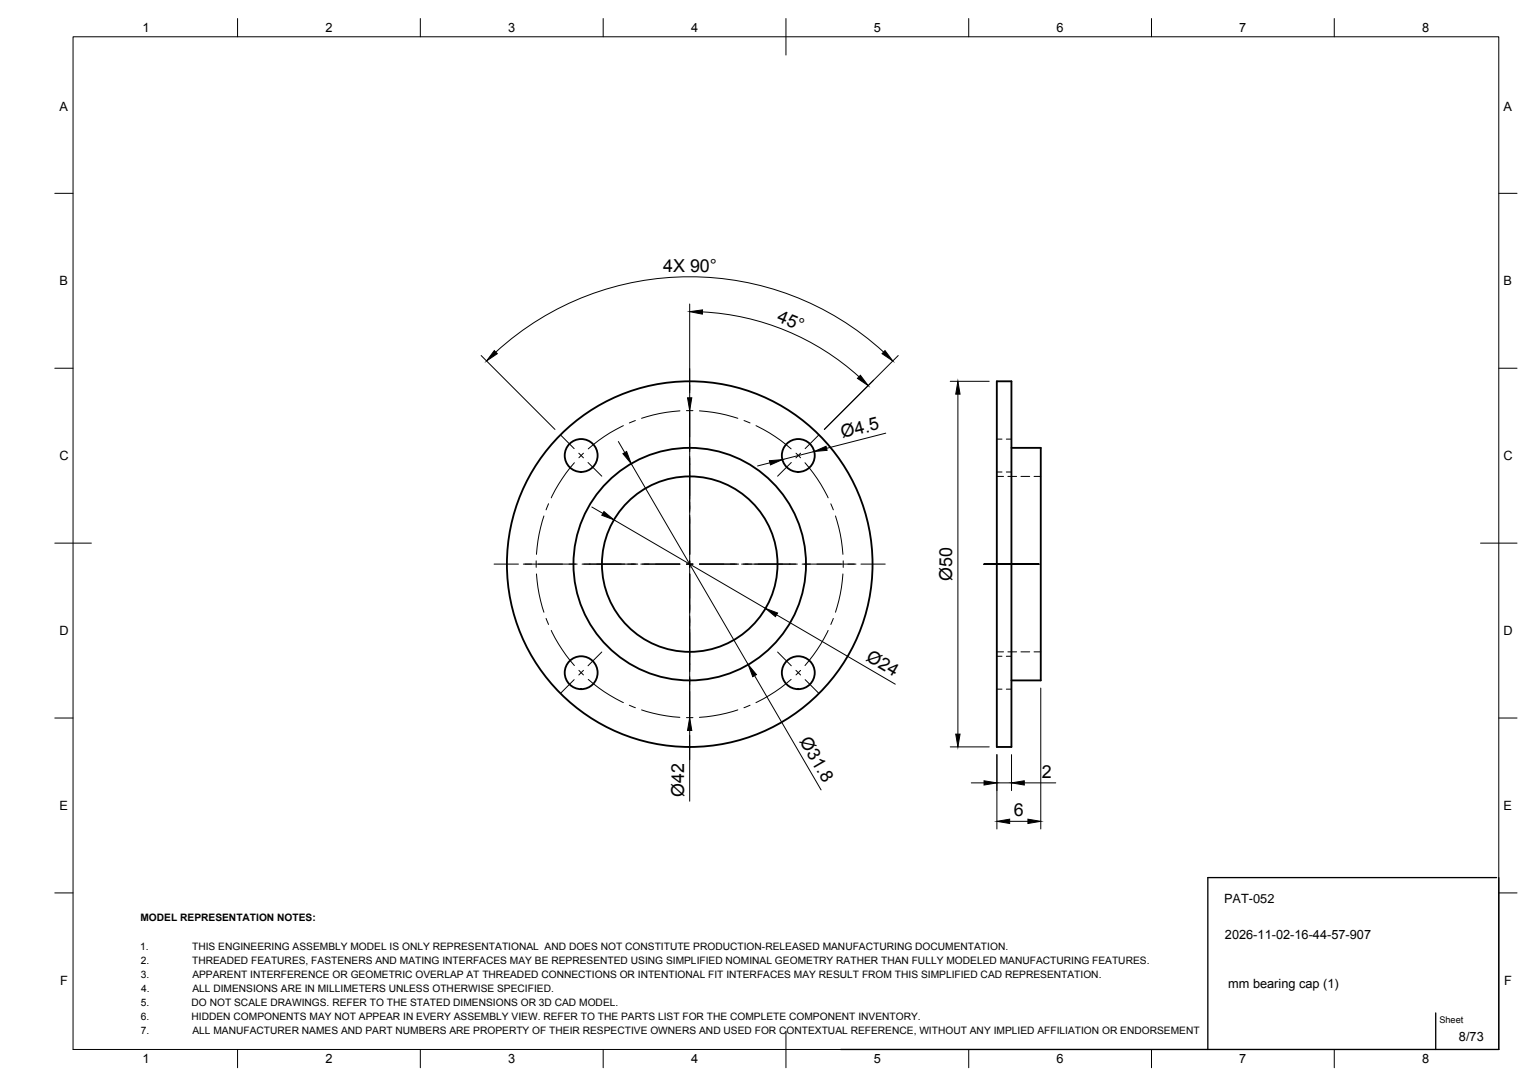
ISO-10303-21;
HEADER;
/* Generated by software containing ST-Developer
 * from STEP Tools, Inc. (www.steptools.com) 
 */

FILE_DESCRIPTION(
/* description */ ('Hand-crank gear train demonstrator'),
/* implementation_level */ '2;1');

FILE_NAME(
/* name */ 'mm bearing cap (1).step',
/* time_stamp */ '2026-10-28T03:22:13-07:00',
/* author */ (''),
/* organization */ (''),
/* preprocessor_version */ 'ST-DEVELOPER v20.2',
/* originating_system */ 'Autodesk Translation Framework v15.17.0.0',
/* authorisation */ '');

FILE_SCHEMA (('AUTOMOTIVE_DESIGN { 1 0 10303 214 3 1 1 }'));
ENDSEC;

DATA;
#10=MECHANICAL_DESIGN_GEOMETRIC_PRESENTATION_REPRESENTATION('',(#1192),#62758);
#1064=SHAPE_REPRESENTATION_RELATIONSHIP('SRR','None',#63036,#1128);
#1128=ADVANCED_BREP_SHAPE_REPRESENTATION('',(#1271),#62690);
#1192=STYLED_ITEM('',(#63462),#1271);
#1271=MANIFOLD_SOLID_BREP('Body1',#16372);
#1409=FACE_BOUND('',#3184,.T.);
#1410=FACE_BOUND('',#3188,.T.);
#1411=FACE_BOUND('',#3189,.T.);
#1412=FACE_BOUND('',#3190,.T.);
#1413=FACE_BOUND('',#3191,.T.);
#1414=FACE_BOUND('',#3192,.T.);
#1415=FACE_BOUND('',#3194,.T.);
#1416=FACE_BOUND('',#3195,.T.);
#1417=FACE_BOUND('',#3196,.T.);
#1418=FACE_BOUND('',#3197,.T.);
#1419=FACE_BOUND('',#3198,.T.);
#1650=PLANE('',#17301);
#1651=PLANE('',#17308);
#1652=PLANE('',#17309);
#2175=FACE_OUTER_BOUND('',#3178,.T.);
#2176=FACE_OUTER_BOUND('',#3179,.T.);
#2177=FACE_OUTER_BOUND('',#3180,.T.);
#2178=FACE_OUTER_BOUND('',#3181,.T.);
#2179=FACE_OUTER_BOUND('',#3182,.T.);
#2180=FACE_OUTER_BOUND('',#3183,.T.);
#2181=FACE_OUTER_BOUND('',#3185,.T.);
#2182=FACE_OUTER_BOUND('',#3186,.T.);
#2183=FACE_OUTER_BOUND('',#3187,.T.);
#2184=FACE_OUTER_BOUND('',#3193,.T.);
#3178=EDGE_LOOP('',(#11105,#11106,#11107,#11108));
#3179=EDGE_LOOP('',(#11109,#11110,#11111,#11112));
#3180=EDGE_LOOP('',(#11113,#11114,#11115,#11116));
#3181=EDGE_LOOP('',(#11117,#11118,#11119,#11120));
#3182=EDGE_LOOP('',(#11121,#11122,#11123,#11124));
#3183=EDGE_LOOP('',(#11125));
#3184=EDGE_LOOP('',(#11126));
#3185=EDGE_LOOP('',(#11127,#11128,#11129,#11130));
#3186=EDGE_LOOP('',(#11131,#11132,#11133,#11134));
#3187=EDGE_LOOP('',(#11135));
#3188=EDGE_LOOP('',(#11136));
#3189=EDGE_LOOP('',(#11137));
#3190=EDGE_LOOP('',(#11138));
#3191=EDGE_LOOP('',(#11139));
#3192=EDGE_LOOP('',(#11140));
#3193=EDGE_LOOP('',(#11141));
#3194=EDGE_LOOP('',(#11142));
#3195=EDGE_LOOP('',(#11143));
#3196=EDGE_LOOP('',(#11144));
#3197=EDGE_LOOP('',(#11145));
#3198=EDGE_LOOP('',(#11146));
#4351=LINE('',#23596,#5483);
#4352=LINE('',#23602,#5484);
#4353=LINE('',#23608,#5485);
#4354=LINE('',#23614,#5486);
#4355=LINE('',#23620,#5487);
#4356=LINE('',#23628,#5488);
#4357=LINE('',#23633,#5489);
#5483=VECTOR('',#19156,0.225);
#5484=VECTOR('',#19163,0.225);
#5485=VECTOR('',#19170,0.225);
#5486=VECTOR('',#19177,0.225);
#5487=VECTOR('',#19184,1.59);
#5488=VECTOR('',#19195,1.2);
#5489=VECTOR('',#19200,2.5);
#6620=CIRCLE('',#17287,0.225);
#6621=CIRCLE('',#17288,0.225);
#6622=CIRCLE('',#17290,0.225);
#6623=CIRCLE('',#17291,0.225);
#6624=CIRCLE('',#17293,0.225);
#6625=CIRCLE('',#17294,0.225);
#6626=CIRCLE('',#17296,0.225);
#6627=CIRCLE('',#17297,0.225);
#6628=CIRCLE('',#17299,1.59);
#6629=CIRCLE('',#17300,1.59);
#6630=CIRCLE('',#17302,1.2);
#6631=CIRCLE('',#17304,1.2);
#6632=CIRCLE('',#17306,2.5);
#6633=CIRCLE('',#17307,2.5);
#7302=VERTEX_POINT('',#23593);
#7303=VERTEX_POINT('',#23595);
#7304=VERTEX_POINT('',#23599);
#7305=VERTEX_POINT('',#23601);
#7306=VERTEX_POINT('',#23605);
#7307=VERTEX_POINT('',#23607);
#7308=VERTEX_POINT('',#23611);
#7309=VERTEX_POINT('',#23613);
#7310=VERTEX_POINT('',#23617);
#7311=VERTEX_POINT('',#23619);
#7312=VERTEX_POINT('',#23623);
#7313=VERTEX_POINT('',#23626);
#7314=VERTEX_POINT('',#23630);
#7315=VERTEX_POINT('',#23632);
#8804=EDGE_CURVE('',#7302,#7302,#6620,.T.);
#8805=EDGE_CURVE('',#7302,#7303,#4351,.T.);
#8806=EDGE_CURVE('',#7303,#7303,#6621,.T.);
#8807=EDGE_CURVE('',#7304,#7304,#6622,.T.);
#8808=EDGE_CURVE('',#7304,#7305,#4352,.T.);
#8809=EDGE_CURVE('',#7305,#7305,#6623,.T.);
#8810=EDGE_CURVE('',#7306,#7306,#6624,.T.);
#8811=EDGE_CURVE('',#7306,#7307,#4353,.T.);
#8812=EDGE_CURVE('',#7307,#7307,#6625,.T.);
#8813=EDGE_CURVE('',#7308,#7308,#6626,.T.);
#8814=EDGE_CURVE('',#7308,#7309,#4354,.T.);
#8815=EDGE_CURVE('',#7309,#7309,#6627,.T.);
#8816=EDGE_CURVE('',#7310,#7310,#6628,.T.);
#8817=EDGE_CURVE('',#7310,#7311,#4355,.T.);
#8818=EDGE_CURVE('',#7311,#7311,#6629,.T.);
#8819=EDGE_CURVE('',#7312,#7312,#6630,.T.);
#8820=EDGE_CURVE('',#7313,#7313,#6631,.T.);
#8821=EDGE_CURVE('',#7313,#7312,#4356,.T.);
#8822=EDGE_CURVE('',#7314,#7314,#6632,.T.);
#8823=EDGE_CURVE('',#7314,#7315,#4357,.T.);
#8824=EDGE_CURVE('',#7315,#7315,#6633,.T.);
#11105=ORIENTED_EDGE('',*,*,#8804,.F.);
#11106=ORIENTED_EDGE('',*,*,#8805,.T.);
#11107=ORIENTED_EDGE('',*,*,#8806,.F.);
#11108=ORIENTED_EDGE('',*,*,#8805,.F.);
#11109=ORIENTED_EDGE('',*,*,#8807,.F.);
#11110=ORIENTED_EDGE('',*,*,#8808,.T.);
#11111=ORIENTED_EDGE('',*,*,#8809,.F.);
#11112=ORIENTED_EDGE('',*,*,#8808,.F.);
#11113=ORIENTED_EDGE('',*,*,#8810,.F.);
#11114=ORIENTED_EDGE('',*,*,#8811,.T.);
#11115=ORIENTED_EDGE('',*,*,#8812,.F.);
#11116=ORIENTED_EDGE('',*,*,#8811,.F.);
#11117=ORIENTED_EDGE('',*,*,#8813,.F.);
#11118=ORIENTED_EDGE('',*,*,#8814,.T.);
#11119=ORIENTED_EDGE('',*,*,#8815,.F.);
#11120=ORIENTED_EDGE('',*,*,#8814,.F.);
#11121=ORIENTED_EDGE('',*,*,#8816,.F.);
#11122=ORIENTED_EDGE('',*,*,#8817,.T.);
#11123=ORIENTED_EDGE('',*,*,#8818,.T.);
#11124=ORIENTED_EDGE('',*,*,#8817,.F.);
#11125=ORIENTED_EDGE('',*,*,#8818,.F.);
#11126=ORIENTED_EDGE('',*,*,#8819,.F.);
#11127=ORIENTED_EDGE('',*,*,#8820,.F.);
#11128=ORIENTED_EDGE('',*,*,#8821,.T.);
#11129=ORIENTED_EDGE('',*,*,#8819,.T.);
#11130=ORIENTED_EDGE('',*,*,#8821,.F.);
#11131=ORIENTED_EDGE('',*,*,#8822,.F.);
#11132=ORIENTED_EDGE('',*,*,#8823,.T.);
#11133=ORIENTED_EDGE('',*,*,#8824,.T.);
#11134=ORIENTED_EDGE('',*,*,#8823,.F.);
#11135=ORIENTED_EDGE('',*,*,#8822,.T.);
#11136=ORIENTED_EDGE('',*,*,#8820,.T.);
#11137=ORIENTED_EDGE('',*,*,#8815,.T.);
#11138=ORIENTED_EDGE('',*,*,#8812,.T.);
#11139=ORIENTED_EDGE('',*,*,#8809,.T.);
#11140=ORIENTED_EDGE('',*,*,#8806,.T.);
#11141=ORIENTED_EDGE('',*,*,#8824,.F.);
#11142=ORIENTED_EDGE('',*,*,#8816,.T.);
#11143=ORIENTED_EDGE('',*,*,#8813,.T.);
#11144=ORIENTED_EDGE('',*,*,#8810,.T.);
#11145=ORIENTED_EDGE('',*,*,#8807,.T.);
#11146=ORIENTED_EDGE('',*,*,#8804,.T.);
#15202=CYLINDRICAL_SURFACE('',#17286,0.225);
#15203=CYLINDRICAL_SURFACE('',#17289,0.225);
#15204=CYLINDRICAL_SURFACE('',#17292,0.225);
#15205=CYLINDRICAL_SURFACE('',#17295,0.225);
#15206=CYLINDRICAL_SURFACE('',#17298,1.59);
#15207=CYLINDRICAL_SURFACE('',#17303,1.2);
#15208=CYLINDRICAL_SURFACE('',#17305,2.5);
#15485=ADVANCED_FACE('',(#2175),#15202,.F.);
#15486=ADVANCED_FACE('',(#2176),#15203,.F.);
#15487=ADVANCED_FACE('',(#2177),#15204,.F.);
#15488=ADVANCED_FACE('',(#2178),#15205,.F.);
#15489=ADVANCED_FACE('',(#2179),#15206,.T.);
#15490=ADVANCED_FACE('',(#2180,#1409),#1650,.F.);
#15491=ADVANCED_FACE('',(#2181),#15207,.F.);
#15492=ADVANCED_FACE('',(#2182),#15208,.T.);
#15493=ADVANCED_FACE('',(#2183,#1410,#1411,#1412,#1413,#1414),#1651,.T.);
#15494=ADVANCED_FACE('',(#2184,#1415,#1416,#1417,#1418,#1419),#1652,.F.);
#16372=CLOSED_SHELL('',(#15485,#15486,#15487,#15488,#15489,#15490,#15491,
#15492,#15493,#15494));
#17285=AXIS2_PLACEMENT_3D('',#23591,#19150,#19151);
#17286=AXIS2_PLACEMENT_3D('',#23592,#19152,#19153);
#17287=AXIS2_PLACEMENT_3D('',#23594,#19154,#19155);
#17288=AXIS2_PLACEMENT_3D('',#23597,#19157,#19158);
#17289=AXIS2_PLACEMENT_3D('',#23598,#19159,#19160);
#17290=AXIS2_PLACEMENT_3D('',#23600,#19161,#19162);
#17291=AXIS2_PLACEMENT_3D('',#23603,#19164,#19165);
#17292=AXIS2_PLACEMENT_3D('',#23604,#19166,#19167);
#17293=AXIS2_PLACEMENT_3D('',#23606,#19168,#19169);
#17294=AXIS2_PLACEMENT_3D('',#23609,#19171,#19172);
#17295=AXIS2_PLACEMENT_3D('',#23610,#19173,#19174);
#17296=AXIS2_PLACEMENT_3D('',#23612,#19175,#19176);
#17297=AXIS2_PLACEMENT_3D('',#23615,#19178,#19179);
#17298=AXIS2_PLACEMENT_3D('',#23616,#19180,#19181);
#17299=AXIS2_PLACEMENT_3D('',#23618,#19182,#19183);
#17300=AXIS2_PLACEMENT_3D('',#23621,#19185,#19186);
#17301=AXIS2_PLACEMENT_3D('',#23622,#19187,#19188);
#17302=AXIS2_PLACEMENT_3D('',#23624,#19189,#19190);
#17303=AXIS2_PLACEMENT_3D('',#23625,#19191,#19192);
#17304=AXIS2_PLACEMENT_3D('',#23627,#19193,#19194);
#17305=AXIS2_PLACEMENT_3D('',#23629,#19196,#19197);
#17306=AXIS2_PLACEMENT_3D('',#23631,#19198,#19199);
#17307=AXIS2_PLACEMENT_3D('',#23634,#19201,#19202);
#17308=AXIS2_PLACEMENT_3D('',#23635,#19203,#19204);
#17309=AXIS2_PLACEMENT_3D('',#23636,#19205,#19206);
#19150=DIRECTION('axis',(0.,0.,1.));
#19151=DIRECTION('refdir',(1.,0.,0.));
#19152=DIRECTION('center_axis',(0.,1.,0.));
#19153=DIRECTION('ref_axis',(1.,0.,0.));
#19154=DIRECTION('center_axis',(0.,1.,0.));
#19155=DIRECTION('ref_axis',(1.,0.,0.));
#19156=DIRECTION('',(0.,1.,0.));
#19157=DIRECTION('center_axis',(0.,-1.,0.));
#19158=DIRECTION('ref_axis',(1.,0.,0.));
#19159=DIRECTION('center_axis',(0.,1.,0.));
#19160=DIRECTION('ref_axis',(1.,0.,0.));
#19161=DIRECTION('center_axis',(0.,1.,0.));
#19162=DIRECTION('ref_axis',(1.,0.,0.));
#19163=DIRECTION('',(0.,1.,0.));
#19164=DIRECTION('center_axis',(0.,-1.,0.));
#19165=DIRECTION('ref_axis',(1.,0.,0.));
#19166=DIRECTION('center_axis',(0.,1.,0.));
#19167=DIRECTION('ref_axis',(1.,0.,0.));
#19168=DIRECTION('center_axis',(0.,1.,0.));
#19169=DIRECTION('ref_axis',(1.,0.,0.));
#19170=DIRECTION('',(0.,1.,0.));
#19171=DIRECTION('center_axis',(0.,-1.,0.));
#19172=DIRECTION('ref_axis',(1.,0.,0.));
#19173=DIRECTION('center_axis',(0.,1.,0.));
#19174=DIRECTION('ref_axis',(1.,0.,0.));
#19175=DIRECTION('center_axis',(0.,1.,0.));
#19176=DIRECTION('ref_axis',(1.,0.,0.));
#19177=DIRECTION('',(0.,1.,0.));
#19178=DIRECTION('center_axis',(0.,-1.,0.));
#19179=DIRECTION('ref_axis',(1.,0.,0.));
#19180=DIRECTION('center_axis',(0.,1.,0.));
#19181=DIRECTION('ref_axis',(1.,0.,0.));
#19182=DIRECTION('center_axis',(0.,1.,0.));
#19183=DIRECTION('ref_axis',(1.,0.,0.));
#19184=DIRECTION('',(0.,-1.,0.));
#19185=DIRECTION('center_axis',(0.,1.,0.));
#19186=DIRECTION('ref_axis',(1.,0.,0.));
#19187=DIRECTION('center_axis',(0.,1.,0.));
#19188=DIRECTION('ref_axis',(1.,0.,0.));
#19189=DIRECTION('center_axis',(0.,-1.,0.));
#19190=DIRECTION('ref_axis',(1.,0.,0.));
#19191=DIRECTION('center_axis',(0.,1.,0.));
#19192=DIRECTION('ref_axis',(1.,0.,0.));
#19193=DIRECTION('center_axis',(0.,-1.,0.));
#19194=DIRECTION('ref_axis',(1.,0.,0.));
#19195=DIRECTION('',(0.,-1.,0.));
#19196=DIRECTION('center_axis',(0.,1.,0.));
#19197=DIRECTION('ref_axis',(1.,0.,0.));
#19198=DIRECTION('center_axis',(0.,1.,0.));
#19199=DIRECTION('ref_axis',(1.,0.,0.));
#19200=DIRECTION('',(0.,-1.,0.));
#19201=DIRECTION('center_axis',(0.,1.,0.));
#19202=DIRECTION('ref_axis',(1.,0.,0.));
#19203=DIRECTION('center_axis',(0.,1.,0.));
#19204=DIRECTION('ref_axis',(1.,0.,0.));
#19205=DIRECTION('center_axis',(0.,1.,0.));
#19206=DIRECTION('ref_axis',(1.,0.,0.));
#23591=CARTESIAN_POINT('',(0.,0.,0.));
#23592=CARTESIAN_POINT('Origin',(-1.48492424049175,-0.7,7.51507575950825));
#23593=CARTESIAN_POINT('',(-1.70992424049175,-0.6,7.51507575950825));
#23594=CARTESIAN_POINT('Origin',(-1.48492424049175,-0.6,7.51507575950825));
#23595=CARTESIAN_POINT('',(-1.70992424049175,-0.4,7.51507575950825));
#23596=CARTESIAN_POINT('',(-1.70992424049175,-0.7,7.51507575950825));
#23597=CARTESIAN_POINT('Origin',(-1.48492424049175,-0.4,7.51507575950825));
#23598=CARTESIAN_POINT('Origin',(-1.48492424049175,-0.7,10.4849242404918));
#23599=CARTESIAN_POINT('',(-1.70992424049175,-0.6,10.4849242404918));
#23600=CARTESIAN_POINT('Origin',(-1.48492424049175,-0.6,10.4849242404918));
#23601=CARTESIAN_POINT('',(-1.70992424049175,-0.4,10.4849242404918));
#23602=CARTESIAN_POINT('',(-1.70992424049175,-0.7,10.4849242404918));
#23603=CARTESIAN_POINT('Origin',(-1.48492424049175,-0.4,10.4849242404918));
#23604=CARTESIAN_POINT('Origin',(1.48492424049175,-0.7,10.4849242404918));
#23605=CARTESIAN_POINT('',(1.25992424049175,-0.6,10.4849242404918));
#23606=CARTESIAN_POINT('Origin',(1.48492424049175,-0.6,10.4849242404918));
#23607=CARTESIAN_POINT('',(1.25992424049175,-0.4,10.4849242404918));
#23608=CARTESIAN_POINT('',(1.25992424049175,-0.7,10.4849242404918));
#23609=CARTESIAN_POINT('Origin',(1.48492424049175,-0.4,10.4849242404918));
#23610=CARTESIAN_POINT('Origin',(1.48492424049175,-0.7,7.51507575950825));
#23611=CARTESIAN_POINT('',(1.25992424049175,-0.6,7.51507575950825));
#23612=CARTESIAN_POINT('Origin',(1.48492424049175,-0.6,7.51507575950825));
#23613=CARTESIAN_POINT('',(1.25992424049175,-0.4,7.51507575950825));
#23614=CARTESIAN_POINT('',(1.25992424049175,-0.7,7.51507575950825));
#23615=CARTESIAN_POINT('Origin',(1.48492424049175,-0.4,7.51507575950825));
#23616=CARTESIAN_POINT('Origin',(0.,-1.,9.));
#23617=CARTESIAN_POINT('',(-1.59,-0.6,9.));
#23618=CARTESIAN_POINT('Origin',(0.,-0.6,9.));
#23619=CARTESIAN_POINT('',(-1.59,-1.,9.));
#23620=CARTESIAN_POINT('',(-1.59,-1.,9.));
#23621=CARTESIAN_POINT('Origin',(0.,-1.,9.));
#23622=CARTESIAN_POINT('Origin',(0.,-1.,9.));
#23623=CARTESIAN_POINT('',(-1.2,-1.,9.));
#23624=CARTESIAN_POINT('Origin',(0.,-1.,9.));
#23625=CARTESIAN_POINT('Origin',(0.,-0.6,9.));
#23626=CARTESIAN_POINT('',(-1.2,-0.4,9.));
#23627=CARTESIAN_POINT('Origin',(0.,-0.4,9.));
#23628=CARTESIAN_POINT('',(-1.2,-0.6,9.));
#23629=CARTESIAN_POINT('Origin',(0.,-0.6,9.));
#23630=CARTESIAN_POINT('',(-2.5,-0.4,9.));
#23631=CARTESIAN_POINT('Origin',(0.,-0.4,9.));
#23632=CARTESIAN_POINT('',(-2.5,-0.6,9.));
#23633=CARTESIAN_POINT('',(-2.5,-0.6,9.));
#23634=CARTESIAN_POINT('Origin',(0.,-0.6,9.));
#23635=CARTESIAN_POINT('Origin',(0.,-0.4,9.));
#23636=CARTESIAN_POINT('Origin',(0.,-0.6,9.));
#62616=UNCERTAINTY_MEASURE_WITH_UNIT(LENGTH_MEASURE(0.001),#62759,
'DISTANCE_ACCURACY_VALUE',
'Maximum model space distance between geometric entities at asserted c
onnectivities');
#62684=UNCERTAINTY_MEASURE_WITH_UNIT(LENGTH_MEASURE(0.001),#62759,
'DISTANCE_ACCURACY_VALUE',
'Maximum model space distance between geometric entities at asserted c
onnectivities');
#62690=(
GEOMETRIC_REPRESENTATION_CONTEXT(3)
GLOBAL_UNCERTAINTY_ASSIGNED_CONTEXT((#62616))
GLOBAL_UNIT_ASSIGNED_CONTEXT((#62759,#62761,#62762))
REPRESENTATION_CONTEXT('','3D')
);
#62758=(
GEOMETRIC_REPRESENTATION_CONTEXT(3)
GLOBAL_UNCERTAINTY_ASSIGNED_CONTEXT((#62684))
GLOBAL_UNIT_ASSIGNED_CONTEXT((#62759,#62761,#62762))
REPRESENTATION_CONTEXT('','3D')
);
#62759=(
LENGTH_UNIT()
NAMED_UNIT(*)
SI_UNIT(.CENTI.,.METRE.)
);
#62761=(
NAMED_UNIT(*)
PLANE_ANGLE_UNIT()
SI_UNIT($,.RADIAN.)
);
#62762=(
NAMED_UNIT(*)
SI_UNIT($,.STERADIAN.)
SOLID_ANGLE_UNIT()
);
#62768=SHAPE_DEFINITION_REPRESENTATION(#62841,#63036);
#62841=PRODUCT_DEFINITION_SHAPE('',$,#63110);
#63036=SHAPE_REPRESENTATION('',(#17285),#62690);
#63104=PRODUCT_DEFINITION_CONTEXT('part definition',#63325,'design');
#63110=PRODUCT_DEFINITION('mm bearing cap (1)','mm bearing cap (1)',#63183,
#63104);
#63183=PRODUCT_DEFINITION_FORMATION('',$,#63332);
#63325=APPLICATION_CONTEXT(
'Core Data for Automotive Mechanical Design Process');
#63326=PRODUCT_CONTEXT('part definition',#63325,'mechanical');
#63332=PRODUCT('mm bearing cap (1)','mm bearing cap (1)','mm bearing cap (1)',
(#63326));
#63456=COLOUR_RGB('Grey',0.48,0.52,0.57);
#63457=FILL_AREA_STYLE_COLOUR('',#63456);
#63458=FILL_AREA_STYLE('',(#63457));
#63459=SURFACE_STYLE_FILL_AREA(#63458);
#63460=SURFACE_SIDE_STYLE('',(#63459));
#63461=SURFACE_STYLE_USAGE(.BOTH.,#63460);
#63462=PRESENTATION_STYLE_ASSIGNMENT((#63461));
ENDSEC;
END-ISO-10303-21;
